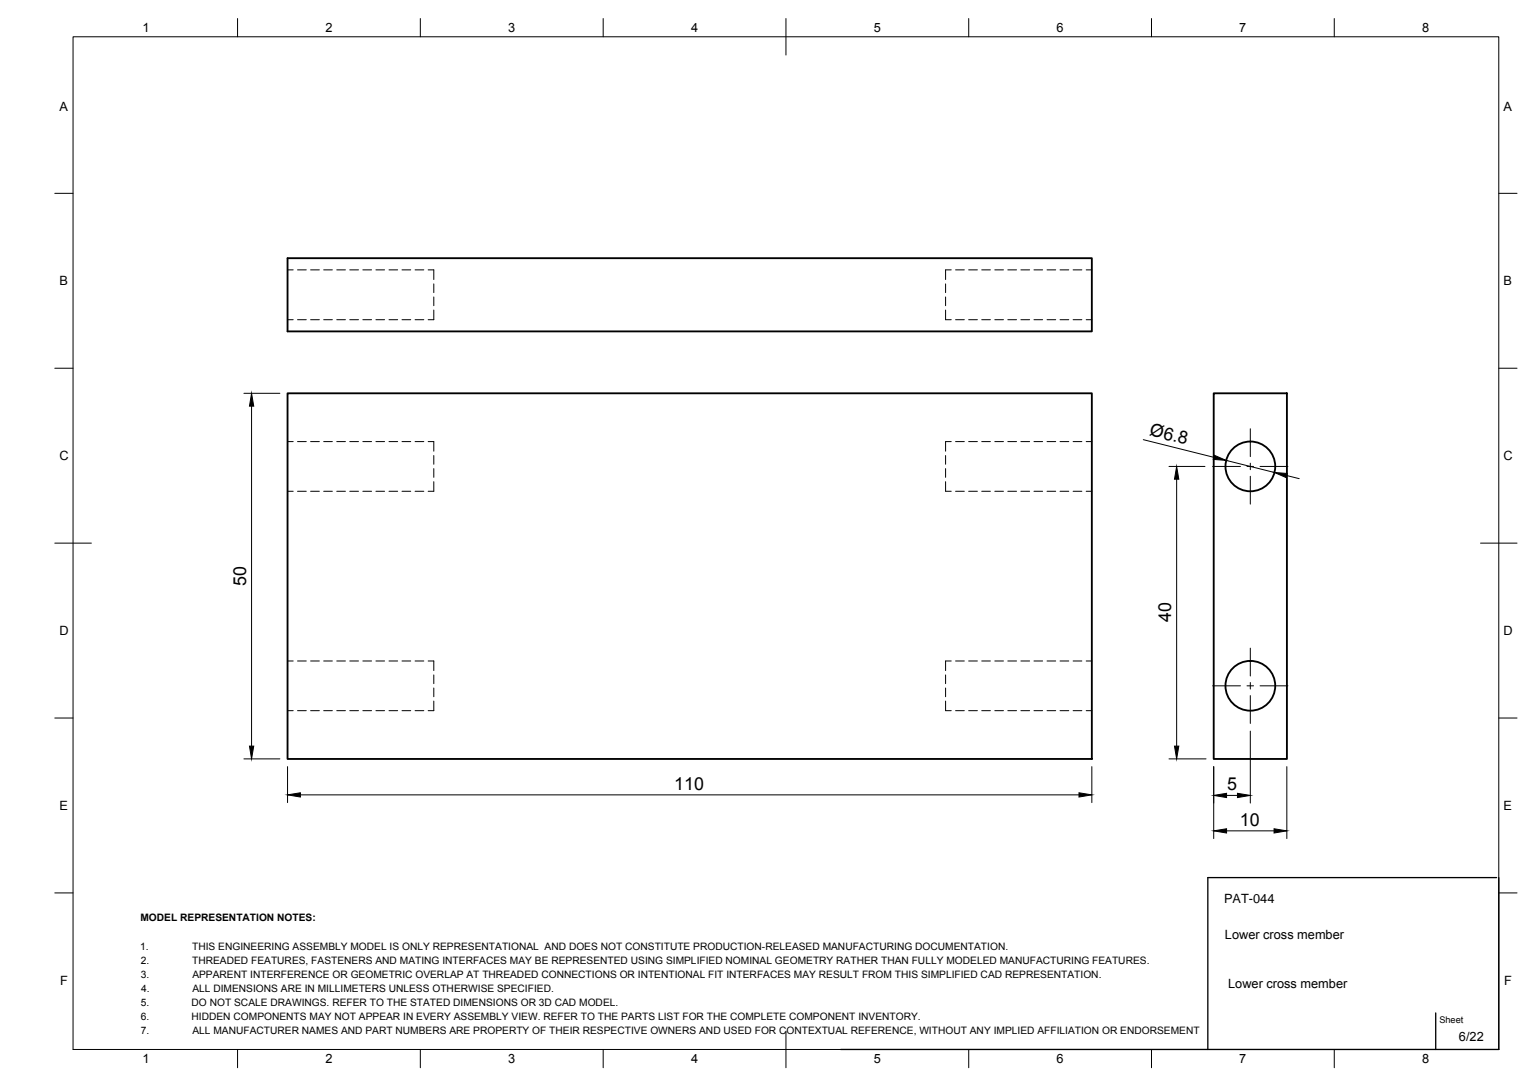
ISO-10303-21;
HEADER;
/* Generated by software containing ST-Developer
 * from STEP Tools, Inc. (www.steptools.com) 
 */

FILE_DESCRIPTION(
/* description */ ('Four-wheel beam trolley'),
/* implementation_level */ '2;1');

FILE_NAME(
/* name */ 'Lower cross member.step',
/* time_stamp */ '2026-10-29T16:22:06-07:00',
/* author */ (''),
/* organization */ (''),
/* preprocessor_version */ 'ST-DEVELOPER v20.2',
/* originating_system */ 'Autodesk Translation Framework v15.17.0.0',
/* authorisation */ '');

FILE_SCHEMA (('AUTOMOTIVE_DESIGN { 1 0 10303 214 3 1 1 }'));
ENDSEC;

DATA;
#10=MECHANICAL_DESIGN_GEOMETRIC_PRESENTATION_REPRESENTATION('',(#278),#4777);
#244=SHAPE_REPRESENTATION_RELATIONSHIP('SRR','None',#4873,#261);
#261=ADVANCED_BREP_SHAPE_REPRESENTATION('',(#302),#4758);
#278=STYLED_ITEM('',(#5049),#302);
#302=MANIFOLD_SOLID_BREP('Body1',#2365);
#324=FACE_BOUND('',#598,.T.);
#325=FACE_BOUND('',#599,.T.);
#326=FACE_BOUND('',#602,.T.);
#327=FACE_BOUND('',#603,.T.);
#365=PLANE('',#2585);
#366=PLANE('',#2589);
#367=PLANE('',#2593);
#368=PLANE('',#2597);
#369=PLANE('',#2598);
#370=PLANE('',#2599);
#371=PLANE('',#2600);
#372=PLANE('',#2601);
#373=PLANE('',#2602);
#374=PLANE('',#2603);
#442=FACE_OUTER_BOUND('',#589,.T.);
#443=FACE_OUTER_BOUND('',#590,.T.);
#444=FACE_OUTER_BOUND('',#591,.T.);
#445=FACE_OUTER_BOUND('',#592,.T.);
#446=FACE_OUTER_BOUND('',#593,.T.);
#447=FACE_OUTER_BOUND('',#594,.T.);
#448=FACE_OUTER_BOUND('',#595,.T.);
#449=FACE_OUTER_BOUND('',#596,.T.);
#450=FACE_OUTER_BOUND('',#597,.T.);
#451=FACE_OUTER_BOUND('',#600,.T.);
#452=FACE_OUTER_BOUND('',#601,.T.);
#453=FACE_OUTER_BOUND('',#604,.T.);
#454=FACE_OUTER_BOUND('',#605,.T.);
#455=FACE_OUTER_BOUND('',#606,.T.);
#589=EDGE_LOOP('',(#1625,#1626,#1627,#1628));
#590=EDGE_LOOP('',(#1629));
#591=EDGE_LOOP('',(#1630,#1631,#1632,#1633));
#592=EDGE_LOOP('',(#1634));
#593=EDGE_LOOP('',(#1635,#1636,#1637,#1638));
#594=EDGE_LOOP('',(#1639));
#595=EDGE_LOOP('',(#1640,#1641,#1642,#1643));
#596=EDGE_LOOP('',(#1644));
#597=EDGE_LOOP('',(#1645,#1646,#1647,#1648));
#598=EDGE_LOOP('',(#1649));
#599=EDGE_LOOP('',(#1650));
#600=EDGE_LOOP('',(#1651,#1652,#1653,#1654));
#601=EDGE_LOOP('',(#1655,#1656,#1657,#1658));
#602=EDGE_LOOP('',(#1659));
#603=EDGE_LOOP('',(#1660));
#604=EDGE_LOOP('',(#1661,#1662,#1663,#1664));
#605=EDGE_LOOP('',(#1665,#1666,#1667,#1668));
#606=EDGE_LOOP('',(#1669,#1670,#1671,#1672));
#777=LINE('',#3768,#900);
#778=LINE('',#3775,#901);
#779=LINE('',#3782,#902);
#780=LINE('',#3789,#903);
#781=LINE('',#3795,#904);
#782=LINE('',#3797,#905);
#783=LINE('',#3799,#906);
#784=LINE('',#3800,#907);
#785=LINE('',#3803,#908);
#786=LINE('',#3805,#909);
#787=LINE('',#3806,#910);
#788=LINE('',#3809,#911);
#789=LINE('',#3811,#912);
#790=LINE('',#3812,#913);
#791=LINE('',#3814,#914);
#792=LINE('',#3815,#915);
#900=VECTOR('',#2942,0.34);
#901=VECTOR('',#2951,0.34);
#902=VECTOR('',#2960,0.34);
#903=VECTOR('',#2969,0.34);
#904=VECTOR('',#2976,1.);
#905=VECTOR('',#2977,1.);
#906=VECTOR('',#2978,1.);
#907=VECTOR('',#2979,1.);
#908=VECTOR('',#2982,1.);
#909=VECTOR('',#2983,1.);
#910=VECTOR('',#2984,1.);
#911=VECTOR('',#2987,1.);
#912=VECTOR('',#2988,1.);
#913=VECTOR('',#2989,1.);
#914=VECTOR('',#2992,1.);
#915=VECTOR('',#2993,1.);
#1023=CIRCLE('',#2583,0.34);
#1024=CIRCLE('',#2584,0.34);
#1025=CIRCLE('',#2587,0.34);
#1026=CIRCLE('',#2588,0.34);
#1027=CIRCLE('',#2591,0.34);
#1028=CIRCLE('',#2592,0.34);
#1029=CIRCLE('',#2595,0.34);
#1030=CIRCLE('',#2596,0.34);
#1161=VERTEX_POINT('',#3765);
#1162=VERTEX_POINT('',#3767);
#1163=VERTEX_POINT('',#3772);
#1164=VERTEX_POINT('',#3774);
#1165=VERTEX_POINT('',#3779);
#1166=VERTEX_POINT('',#3781);
#1167=VERTEX_POINT('',#3786);
#1168=VERTEX_POINT('',#3788);
#1169=VERTEX_POINT('',#3793);
#1170=VERTEX_POINT('',#3794);
#1171=VERTEX_POINT('',#3796);
#1172=VERTEX_POINT('',#3798);
#1173=VERTEX_POINT('',#3802);
#1174=VERTEX_POINT('',#3804);
#1175=VERTEX_POINT('',#3808);
#1176=VERTEX_POINT('',#3810);
#1350=EDGE_CURVE('',#1161,#1161,#1023,.T.);
#1351=EDGE_CURVE('',#1161,#1162,#777,.T.);
#1352=EDGE_CURVE('',#1162,#1162,#1024,.T.);
#1353=EDGE_CURVE('',#1163,#1163,#1025,.T.);
#1354=EDGE_CURVE('',#1163,#1164,#778,.T.);
#1355=EDGE_CURVE('',#1164,#1164,#1026,.T.);
#1356=EDGE_CURVE('',#1165,#1165,#1027,.T.);
#1357=EDGE_CURVE('',#1165,#1166,#779,.T.);
#1358=EDGE_CURVE('',#1166,#1166,#1028,.T.);
#1359=EDGE_CURVE('',#1167,#1167,#1029,.T.);
#1360=EDGE_CURVE('',#1167,#1168,#780,.T.);
#1361=EDGE_CURVE('',#1168,#1168,#1030,.T.);
#1362=EDGE_CURVE('',#1169,#1170,#781,.T.);
#1363=EDGE_CURVE('',#1170,#1171,#782,.T.);
#1364=EDGE_CURVE('',#1172,#1171,#783,.T.);
#1365=EDGE_CURVE('',#1169,#1172,#784,.T.);
#1366=EDGE_CURVE('',#1173,#1169,#785,.T.);
#1367=EDGE_CURVE('',#1174,#1172,#786,.T.);
#1368=EDGE_CURVE('',#1173,#1174,#787,.T.);
#1369=EDGE_CURVE('',#1175,#1173,#788,.T.);
#1370=EDGE_CURVE('',#1176,#1174,#789,.T.);
#1371=EDGE_CURVE('',#1175,#1176,#790,.T.);
#1372=EDGE_CURVE('',#1170,#1175,#791,.T.);
#1373=EDGE_CURVE('',#1171,#1176,#792,.T.);
#1625=ORIENTED_EDGE('',*,*,#1350,.F.);
#1626=ORIENTED_EDGE('',*,*,#1351,.T.);
#1627=ORIENTED_EDGE('',*,*,#1352,.F.);
#1628=ORIENTED_EDGE('',*,*,#1351,.F.);
#1629=ORIENTED_EDGE('',*,*,#1350,.T.);
#1630=ORIENTED_EDGE('',*,*,#1353,.F.);
#1631=ORIENTED_EDGE('',*,*,#1354,.T.);
#1632=ORIENTED_EDGE('',*,*,#1355,.F.);
#1633=ORIENTED_EDGE('',*,*,#1354,.F.);
#1634=ORIENTED_EDGE('',*,*,#1353,.T.);
#1635=ORIENTED_EDGE('',*,*,#1356,.F.);
#1636=ORIENTED_EDGE('',*,*,#1357,.T.);
#1637=ORIENTED_EDGE('',*,*,#1358,.T.);
#1638=ORIENTED_EDGE('',*,*,#1357,.F.);
#1639=ORIENTED_EDGE('',*,*,#1358,.F.);
#1640=ORIENTED_EDGE('',*,*,#1359,.F.);
#1641=ORIENTED_EDGE('',*,*,#1360,.T.);
#1642=ORIENTED_EDGE('',*,*,#1361,.T.);
#1643=ORIENTED_EDGE('',*,*,#1360,.F.);
#1644=ORIENTED_EDGE('',*,*,#1361,.F.);
#1645=ORIENTED_EDGE('',*,*,#1362,.T.);
#1646=ORIENTED_EDGE('',*,*,#1363,.T.);
#1647=ORIENTED_EDGE('',*,*,#1364,.F.);
#1648=ORIENTED_EDGE('',*,*,#1365,.F.);
#1649=ORIENTED_EDGE('',*,*,#1352,.T.);
#1650=ORIENTED_EDGE('',*,*,#1355,.T.);
#1651=ORIENTED_EDGE('',*,*,#1366,.T.);
#1652=ORIENTED_EDGE('',*,*,#1365,.T.);
#1653=ORIENTED_EDGE('',*,*,#1367,.F.);
#1654=ORIENTED_EDGE('',*,*,#1368,.F.);
#1655=ORIENTED_EDGE('',*,*,#1369,.T.);
#1656=ORIENTED_EDGE('',*,*,#1368,.T.);
#1657=ORIENTED_EDGE('',*,*,#1370,.F.);
#1658=ORIENTED_EDGE('',*,*,#1371,.F.);
#1659=ORIENTED_EDGE('',*,*,#1356,.T.);
#1660=ORIENTED_EDGE('',*,*,#1359,.T.);
#1661=ORIENTED_EDGE('',*,*,#1372,.T.);
#1662=ORIENTED_EDGE('',*,*,#1371,.T.);
#1663=ORIENTED_EDGE('',*,*,#1373,.F.);
#1664=ORIENTED_EDGE('',*,*,#1363,.F.);
#1665=ORIENTED_EDGE('',*,*,#1373,.T.);
#1666=ORIENTED_EDGE('',*,*,#1370,.T.);
#1667=ORIENTED_EDGE('',*,*,#1367,.T.);
#1668=ORIENTED_EDGE('',*,*,#1364,.T.);
#1669=ORIENTED_EDGE('',*,*,#1372,.F.);
#1670=ORIENTED_EDGE('',*,*,#1362,.F.);
#1671=ORIENTED_EDGE('',*,*,#1366,.F.);
#1672=ORIENTED_EDGE('',*,*,#1369,.F.);
#2175=CYLINDRICAL_SURFACE('',#2582,0.34);
#2176=CYLINDRICAL_SURFACE('',#2586,0.34);
#2177=CYLINDRICAL_SURFACE('',#2590,0.34);
#2178=CYLINDRICAL_SURFACE('',#2594,0.34);
#2218=ADVANCED_FACE('',(#442),#2175,.F.);
#2219=ADVANCED_FACE('',(#443),#365,.T.);
#2220=ADVANCED_FACE('',(#444),#2176,.F.);
#2221=ADVANCED_FACE('',(#445),#366,.T.);
#2222=ADVANCED_FACE('',(#446),#2177,.F.);
#2223=ADVANCED_FACE('',(#447),#367,.F.);
#2224=ADVANCED_FACE('',(#448),#2178,.F.);
#2225=ADVANCED_FACE('',(#449),#368,.F.);
#2226=ADVANCED_FACE('',(#450,#324,#325),#369,.T.);
#2227=ADVANCED_FACE('',(#451),#370,.T.);
#2228=ADVANCED_FACE('',(#452,#326,#327),#371,.T.);
#2229=ADVANCED_FACE('',(#453),#372,.T.);
#2230=ADVANCED_FACE('',(#454),#373,.T.);
#2231=ADVANCED_FACE('',(#455),#374,.F.);
#2365=CLOSED_SHELL('',(#2218,#2219,#2220,#2221,#2222,#2223,#2224,#2225,
#2226,#2227,#2228,#2229,#2230,#2231));
#2581=AXIS2_PLACEMENT_3D('',#3763,#2936,#2937);
#2582=AXIS2_PLACEMENT_3D('',#3764,#2938,#2939);
#2583=AXIS2_PLACEMENT_3D('',#3766,#2940,#2941);
#2584=AXIS2_PLACEMENT_3D('',#3769,#2943,#2944);
#2585=AXIS2_PLACEMENT_3D('',#3770,#2945,#2946);
#2586=AXIS2_PLACEMENT_3D('',#3771,#2947,#2948);
#2587=AXIS2_PLACEMENT_3D('',#3773,#2949,#2950);
#2588=AXIS2_PLACEMENT_3D('',#3776,#2952,#2953);
#2589=AXIS2_PLACEMENT_3D('',#3777,#2954,#2955);
#2590=AXIS2_PLACEMENT_3D('',#3778,#2956,#2957);
#2591=AXIS2_PLACEMENT_3D('',#3780,#2958,#2959);
#2592=AXIS2_PLACEMENT_3D('',#3783,#2961,#2962);
#2593=AXIS2_PLACEMENT_3D('',#3784,#2963,#2964);
#2594=AXIS2_PLACEMENT_3D('',#3785,#2965,#2966);
#2595=AXIS2_PLACEMENT_3D('',#3787,#2967,#2968);
#2596=AXIS2_PLACEMENT_3D('',#3790,#2970,#2971);
#2597=AXIS2_PLACEMENT_3D('',#3791,#2972,#2973);
#2598=AXIS2_PLACEMENT_3D('',#3792,#2974,#2975);
#2599=AXIS2_PLACEMENT_3D('',#3801,#2980,#2981);
#2600=AXIS2_PLACEMENT_3D('',#3807,#2985,#2986);
#2601=AXIS2_PLACEMENT_3D('',#3813,#2990,#2991);
#2602=AXIS2_PLACEMENT_3D('',#3816,#2994,#2995);
#2603=AXIS2_PLACEMENT_3D('',#3817,#2996,#2997);
#2936=DIRECTION('axis',(0.,0.,1.));
#2937=DIRECTION('refdir',(1.,0.,0.));
#2938=DIRECTION('center_axis',(0.,1.,0.));
#2939=DIRECTION('ref_axis',(1.,0.,0.));
#2940=DIRECTION('center_axis',(0.,1.,0.));
#2941=DIRECTION('ref_axis',(1.,0.,0.));
#2942=DIRECTION('',(0.,1.,0.));
#2943=DIRECTION('center_axis',(0.,-1.,0.));
#2944=DIRECTION('ref_axis',(1.,0.,0.));
#2945=DIRECTION('center_axis',(0.,1.,0.));
#2946=DIRECTION('ref_axis',(1.,0.,0.));
#2947=DIRECTION('center_axis',(0.,1.,0.));
#2948=DIRECTION('ref_axis',(1.,0.,0.));
#2949=DIRECTION('center_axis',(0.,1.,0.));
#2950=DIRECTION('ref_axis',(1.,0.,0.));
#2951=DIRECTION('',(0.,1.,0.));
#2952=DIRECTION('center_axis',(0.,-1.,0.));
#2953=DIRECTION('ref_axis',(1.,0.,0.));
#2954=DIRECTION('center_axis',(0.,1.,0.));
#2955=DIRECTION('ref_axis',(1.,0.,0.));
#2956=DIRECTION('center_axis',(0.,1.,0.));
#2957=DIRECTION('ref_axis',(1.,0.,0.));
#2958=DIRECTION('center_axis',(0.,1.,0.));
#2959=DIRECTION('ref_axis',(1.,0.,0.));
#2960=DIRECTION('',(0.,1.,0.));
#2961=DIRECTION('center_axis',(0.,1.,0.));
#2962=DIRECTION('ref_axis',(1.,0.,0.));
#2963=DIRECTION('center_axis',(0.,1.,0.));
#2964=DIRECTION('ref_axis',(1.,0.,0.));
#2965=DIRECTION('center_axis',(0.,1.,0.));
#2966=DIRECTION('ref_axis',(1.,0.,0.));
#2967=DIRECTION('center_axis',(0.,1.,0.));
#2968=DIRECTION('ref_axis',(1.,0.,0.));
#2969=DIRECTION('',(0.,1.,0.));
#2970=DIRECTION('center_axis',(0.,1.,0.));
#2971=DIRECTION('ref_axis',(1.,0.,0.));
#2972=DIRECTION('center_axis',(0.,1.,0.));
#2973=DIRECTION('ref_axis',(1.,0.,0.));
#2974=DIRECTION('center_axis',(0.,1.,0.));
#2975=DIRECTION('ref_axis',(-1.,0.,0.));
#2976=DIRECTION('',(-1.,0.,0.));
#2977=DIRECTION('',(0.,0.,1.));
#2978=DIRECTION('',(-1.,0.,0.));
#2979=DIRECTION('',(0.,0.,1.));
#2980=DIRECTION('center_axis',(1.,0.,0.));
#2981=DIRECTION('ref_axis',(0.,1.,0.));
#2982=DIRECTION('',(0.,1.,0.));
#2983=DIRECTION('',(0.,1.,0.));
#2984=DIRECTION('',(0.,0.,1.));
#2985=DIRECTION('center_axis',(0.,-1.,0.));
#2986=DIRECTION('ref_axis',(1.,0.,0.));
#2987=DIRECTION('',(1.,0.,0.));
#2988=DIRECTION('',(1.,0.,0.));
#2989=DIRECTION('',(0.,0.,1.));
#2990=DIRECTION('center_axis',(-1.,0.,0.));
#2991=DIRECTION('ref_axis',(0.,-1.,0.));
#2992=DIRECTION('',(0.,-1.,0.));
#2993=DIRECTION('',(0.,-1.,0.));
#2994=DIRECTION('center_axis',(0.,0.,1.));
#2995=DIRECTION('ref_axis',(1.,0.,0.));
#2996=DIRECTION('center_axis',(0.,0.,1.));
#2997=DIRECTION('ref_axis',(1.,0.,0.));
#3763=CARTESIAN_POINT('',(0.,0.,0.));
#3764=CARTESIAN_POINT('Origin',(-1.5,3.5,7.5));
#3765=CARTESIAN_POINT('',(-1.84,3.5,7.5));
#3766=CARTESIAN_POINT('Origin',(-1.5,3.5,7.5));
#3767=CARTESIAN_POINT('',(-1.84,5.5,7.5));
#3768=CARTESIAN_POINT('',(-1.84,3.5,7.5));
#3769=CARTESIAN_POINT('Origin',(-1.5,5.5,7.5));
#3770=CARTESIAN_POINT('Origin',(-1.5,3.5,7.5));
#3771=CARTESIAN_POINT('Origin',(1.5,3.5,7.5));
#3772=CARTESIAN_POINT('',(1.16,3.5,7.5));
#3773=CARTESIAN_POINT('Origin',(1.5,3.5,7.5));
#3774=CARTESIAN_POINT('',(1.16,5.5,7.5));
#3775=CARTESIAN_POINT('',(1.16,3.5,7.5));
#3776=CARTESIAN_POINT('Origin',(1.5,5.5,7.5));
#3777=CARTESIAN_POINT('Origin',(1.5,3.5,7.5));
#3778=CARTESIAN_POINT('Origin',(-1.5,-5.6,7.5));
#3779=CARTESIAN_POINT('',(-1.84,-5.5,7.5));
#3780=CARTESIAN_POINT('Origin',(-1.5,-5.5,7.5));
#3781=CARTESIAN_POINT('',(-1.84,-3.5,7.5));
#3782=CARTESIAN_POINT('',(-1.84,-5.6,7.5));
#3783=CARTESIAN_POINT('Origin',(-1.5,-3.5,7.5));
#3784=CARTESIAN_POINT('Origin',(-1.5,-3.5,7.5));
#3785=CARTESIAN_POINT('Origin',(1.5,-5.6,7.5));
#3786=CARTESIAN_POINT('',(1.16,-5.5,7.5));
#3787=CARTESIAN_POINT('Origin',(1.5,-5.5,7.5));
#3788=CARTESIAN_POINT('',(1.16,-3.5,7.5));
#3789=CARTESIAN_POINT('',(1.16,-5.6,7.5));
#3790=CARTESIAN_POINT('Origin',(1.5,-3.5,7.5));
#3791=CARTESIAN_POINT('Origin',(1.5,-3.5,7.5));
#3792=CARTESIAN_POINT('Origin',(2.5,5.5,7.));
#3793=CARTESIAN_POINT('',(2.5,5.5,7.));
#3794=CARTESIAN_POINT('',(-2.5,5.5,7.));
#3795=CARTESIAN_POINT('',(2.5,5.5,7.));
#3796=CARTESIAN_POINT('',(-2.5,5.5,8.));
#3797=CARTESIAN_POINT('',(-2.5,5.5,7.));
#3798=CARTESIAN_POINT('',(2.5,5.5,8.));
#3799=CARTESIAN_POINT('',(2.5,5.5,8.));
#3800=CARTESIAN_POINT('',(2.5,5.5,7.));
#3801=CARTESIAN_POINT('Origin',(2.5,-5.5,7.));
#3802=CARTESIAN_POINT('',(2.5,-5.5,7.));
#3803=CARTESIAN_POINT('',(2.5,-5.5,7.));
#3804=CARTESIAN_POINT('',(2.5,-5.5,8.));
#3805=CARTESIAN_POINT('',(2.5,-5.5,8.));
#3806=CARTESIAN_POINT('',(2.5,-5.5,7.));
#3807=CARTESIAN_POINT('Origin',(-2.5,-5.5,7.));
#3808=CARTESIAN_POINT('',(-2.5,-5.5,7.));
#3809=CARTESIAN_POINT('',(-2.5,-5.5,7.));
#3810=CARTESIAN_POINT('',(-2.5,-5.5,8.));
#3811=CARTESIAN_POINT('',(-2.5,-5.5,8.));
#3812=CARTESIAN_POINT('',(-2.5,-5.5,7.));
#3813=CARTESIAN_POINT('Origin',(-2.5,5.5,7.));
#3814=CARTESIAN_POINT('',(-2.5,5.5,7.));
#3815=CARTESIAN_POINT('',(-2.5,5.5,8.));
#3816=CARTESIAN_POINT('Origin',(0.,0.,8.));
#3817=CARTESIAN_POINT('Origin',(0.,0.,7.));
#4736=UNCERTAINTY_MEASURE_WITH_UNIT(LENGTH_MEASURE(0.001),#4778,
'DISTANCE_ACCURACY_VALUE',
'Maximum model space distance between geometric entities at asserted c
onnectivities');
#4755=UNCERTAINTY_MEASURE_WITH_UNIT(LENGTH_MEASURE(0.001),#4778,
'DISTANCE_ACCURACY_VALUE',
'Maximum model space distance between geometric entities at asserted c
onnectivities');
#4758=(
GEOMETRIC_REPRESENTATION_CONTEXT(3)
GLOBAL_UNCERTAINTY_ASSIGNED_CONTEXT((#4736))
GLOBAL_UNIT_ASSIGNED_CONTEXT((#4778,#4780,#4781))
REPRESENTATION_CONTEXT('','3D')
);
#4777=(
GEOMETRIC_REPRESENTATION_CONTEXT(3)
GLOBAL_UNCERTAINTY_ASSIGNED_CONTEXT((#4755))
GLOBAL_UNIT_ASSIGNED_CONTEXT((#4778,#4780,#4781))
REPRESENTATION_CONTEXT('','3D')
);
#4778=(
LENGTH_UNIT()
NAMED_UNIT(*)
SI_UNIT(.CENTI.,.METRE.)
);
#4780=(
NAMED_UNIT(*)
PLANE_ANGLE_UNIT()
SI_UNIT($,.RADIAN.)
);
#4781=(
NAMED_UNIT(*)
SI_UNIT($,.STERADIAN.)
SOLID_ANGLE_UNIT()
);
#4784=SHAPE_DEFINITION_REPRESENTATION(#4805,#4873);
#4805=PRODUCT_DEFINITION_SHAPE('',$,#4895);
#4873=SHAPE_REPRESENTATION('',(#2581),#4758);
#4892=PRODUCT_DEFINITION_CONTEXT('part definition',#4957,'design');
#4895=PRODUCT_DEFINITION('Lower cross member','Lower cross member',#4916,
#4892);
#4916=PRODUCT_DEFINITION_FORMATION('',$,#4961);
#4957=APPLICATION_CONTEXT(
'Core Data for Automotive Mechanical Design Process');
#4958=PRODUCT_CONTEXT('part definition',#4957,'mechanical');
#4961=PRODUCT('Lower cross member','Lower cross member',
'Lower cross member',(#4958));
#5043=COLOUR_RGB('Sky Blue',0.24,0.69,0.87);
#5044=FILL_AREA_STYLE_COLOUR('',#5043);
#5045=FILL_AREA_STYLE('',(#5044));
#5046=SURFACE_STYLE_FILL_AREA(#5045);
#5047=SURFACE_SIDE_STYLE('',(#5046));
#5048=SURFACE_STYLE_USAGE(.BOTH.,#5047);
#5049=PRESENTATION_STYLE_ASSIGNMENT((#5048));
ENDSEC;
END-ISO-10303-21;
